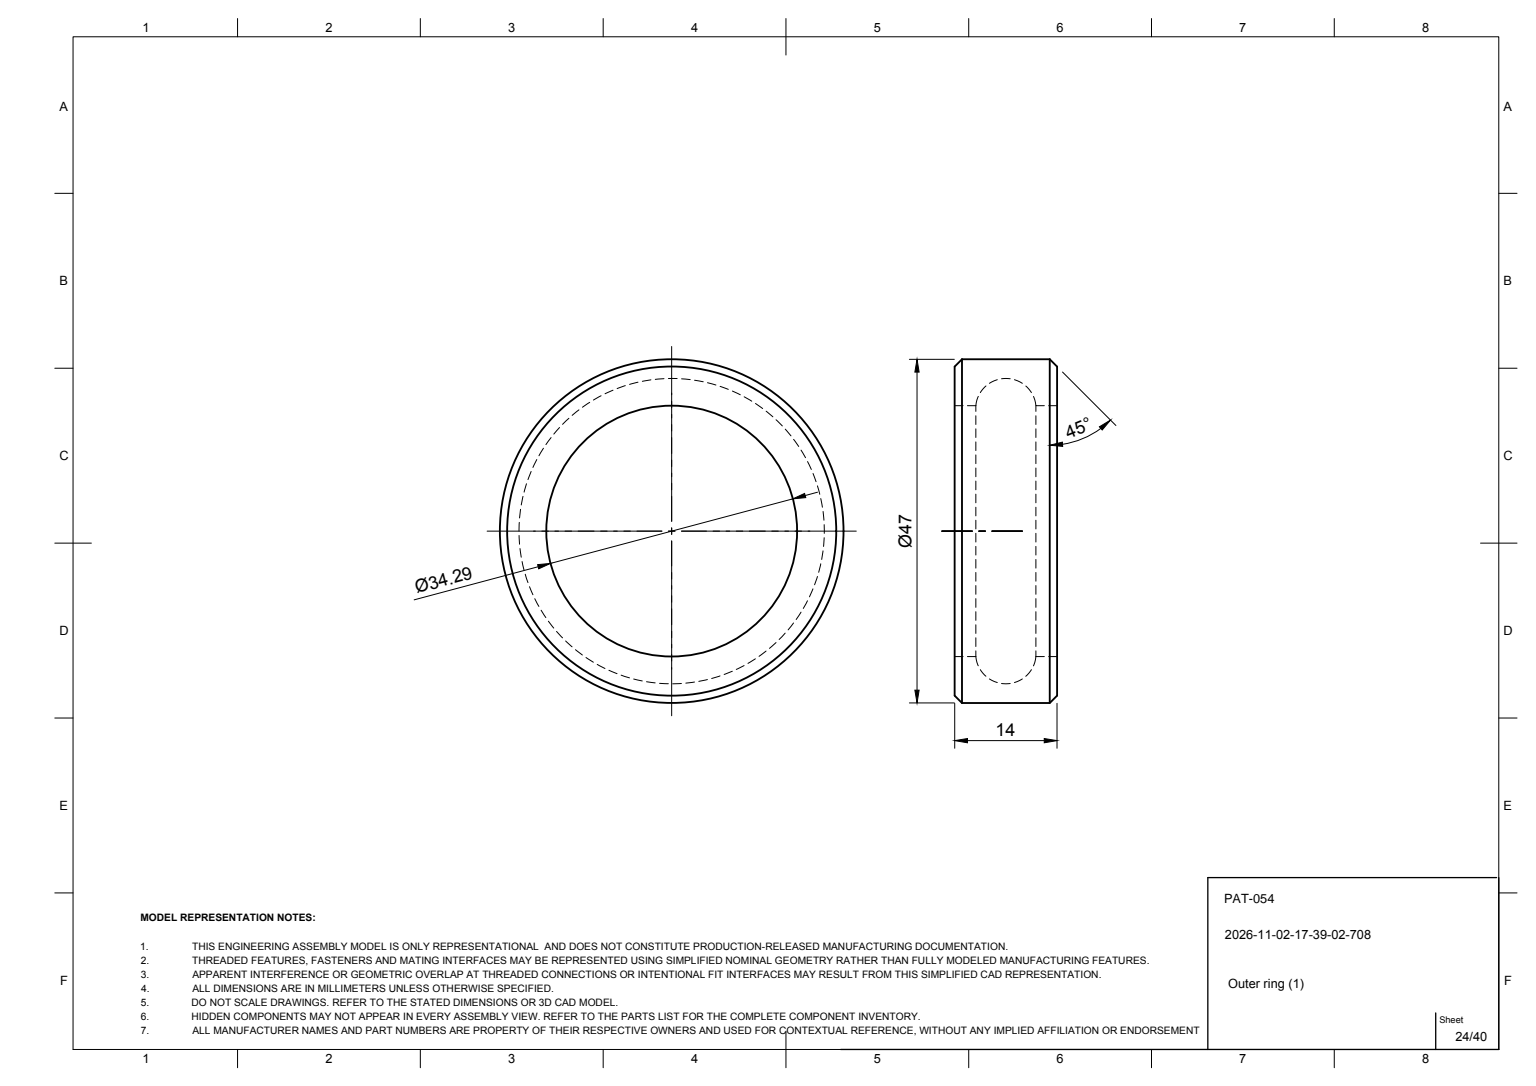
ISO-10303-21;
HEADER;
/* Generated by software containing ST-Developer
 * from STEP Tools, Inc. (www.steptools.com) 
 */

FILE_DESCRIPTION(
/* description */ ('PAT-054'),
/* implementation_level */ '2;1');

FILE_NAME(
/* name */ 'Outer ring (1).step',
/* time_stamp */ '2026-10-29T16:38:13-07:00',
/* author */ (''),
/* organization */ (''),
/* preprocessor_version */ 'ST-DEVELOPER v20.2',
/* originating_system */ 'Autodesk Translation Framework v15.17.0.0',
/* authorisation */ '');

FILE_SCHEMA (('AUTOMOTIVE_DESIGN { 1 0 10303 214 3 1 1 }'));
ENDSEC;

DATA;
#10=MECHANICAL_DESIGN_GEOMETRIC_PRESENTATION_REPRESENTATION('',(#921),#33981);
#783=CONICAL_SURFACE('',#14032,2.3,0.785398163397449);
#784=CONICAL_SURFACE('',#14036,2.3,0.785398163397449);
#810=TOROIDAL_SURFACE('',#14021,1.675,0.412776);
#826=SHAPE_REPRESENTATION_RELATIONSHIP('SRR','None',#34201,#870);
#870=ADVANCED_BREP_SHAPE_REPRESENTATION('',(#980),#33949);
#921=STYLED_ITEM('',(#34517),#980);
#980=MANIFOLD_SOLID_BREP('Body1',#13032);
#1139=FACE_BOUND('',#2637,.T.);
#1140=FACE_BOUND('',#2642,.T.);
#1329=PLANE('',#14029);
#1330=PLANE('',#14038);
#1784=FACE_OUTER_BOUND('',#2634,.T.);
#1785=FACE_OUTER_BOUND('',#2635,.T.);
#1786=FACE_OUTER_BOUND('',#2636,.T.);
#1787=FACE_OUTER_BOUND('',#2638,.T.);
#1788=FACE_OUTER_BOUND('',#2639,.T.);
#1789=FACE_OUTER_BOUND('',#2640,.T.);
#1790=FACE_OUTER_BOUND('',#2641,.T.);
#1791=FACE_OUTER_BOUND('',#2643,.T.);
#2634=EDGE_LOOP('',(#9457,#9458,#9459,#9460,#9461,#9462));
#2635=EDGE_LOOP('',(#9463,#9464,#9465,#9466,#9467));
#2636=EDGE_LOOP('',(#9468));
#2637=EDGE_LOOP('',(#9469));
#2638=EDGE_LOOP('',(#9470,#9471,#9472,#9473));
#2639=EDGE_LOOP('',(#9474,#9475,#9476,#9477));
#2640=EDGE_LOOP('',(#9478,#9479,#9480,#9481));
#2641=EDGE_LOOP('',(#9482));
#2642=EDGE_LOOP('',(#9483));
#2643=EDGE_LOOP('',(#9484,#9485,#9486,#9487,#9488));
#3479=LINE('',#19841,#4413);
#3480=LINE('',#19850,#4414);
#3481=LINE('',#19854,#4415);
#3482=LINE('',#19858,#4416);
#3483=LINE('',#19861,#4417);
#4413=VECTOR('',#16072,1.71469);
#4414=VECTOR('',#16083,2.3);
#4415=VECTOR('',#16088,2.35);
#4416=VECTOR('',#16093,2.3);
#4417=VECTOR('',#16098,1.71469);
#5333=CIRCLE('',#14022,1.71469);
#5334=CIRCLE('',#14023,1.71469);
#5335=CIRCLE('',#14024,0.412776);
#5336=CIRCLE('',#14025,1.71469);
#5337=CIRCLE('',#14026,1.71469);
#5338=CIRCLE('',#14028,1.71469);
#5339=CIRCLE('',#14030,2.25);
#5340=CIRCLE('',#14031,1.71469);
#5341=CIRCLE('',#14033,2.35);
#5342=CIRCLE('',#14035,2.35);
#5343=CIRCLE('',#14037,2.25);
#5900=VERTEX_POINT('',#19829);
#5901=VERTEX_POINT('',#19830);
#5902=VERTEX_POINT('',#19833);
#5903=VERTEX_POINT('',#19835);
#5904=VERTEX_POINT('',#19839);
#5905=VERTEX_POINT('',#19843);
#5906=VERTEX_POINT('',#19845);
#5907=VERTEX_POINT('',#19848);
#5908=VERTEX_POINT('',#19852);
#5909=VERTEX_POINT('',#19856);
#7228=EDGE_CURVE('',#5900,#5901,#5333,.T.);
#7229=EDGE_CURVE('',#5901,#5900,#5334,.T.);
#7230=EDGE_CURVE('',#5901,#5902,#5335,.T.);
#7231=EDGE_CURVE('',#5903,#5902,#5336,.T.);
#7232=EDGE_CURVE('',#5902,#5903,#5337,.T.);
#7233=EDGE_CURVE('',#5904,#5904,#5338,.T.);
#7234=EDGE_CURVE('',#5904,#5903,#3479,.T.);
#7235=EDGE_CURVE('',#5905,#5905,#5339,.T.);
#7236=EDGE_CURVE('',#5906,#5906,#5340,.T.);
#7237=EDGE_CURVE('',#5907,#5907,#5341,.T.);
#7238=EDGE_CURVE('',#5907,#5905,#3480,.T.);
#7239=EDGE_CURVE('',#5908,#5908,#5342,.T.);
#7240=EDGE_CURVE('',#5908,#5907,#3481,.T.);
#7241=EDGE_CURVE('',#5909,#5909,#5343,.T.);
#7242=EDGE_CURVE('',#5909,#5908,#3482,.T.);
#7243=EDGE_CURVE('',#5900,#5906,#3483,.T.);
#9457=ORIENTED_EDGE('',*,*,#7228,.F.);
#9458=ORIENTED_EDGE('',*,*,#7229,.F.);
#9459=ORIENTED_EDGE('',*,*,#7230,.T.);
#9460=ORIENTED_EDGE('',*,*,#7231,.F.);
#9461=ORIENTED_EDGE('',*,*,#7232,.F.);
#9462=ORIENTED_EDGE('',*,*,#7230,.F.);
#9463=ORIENTED_EDGE('',*,*,#7233,.T.);
#9464=ORIENTED_EDGE('',*,*,#7234,.T.);
#9465=ORIENTED_EDGE('',*,*,#7231,.T.);
#9466=ORIENTED_EDGE('',*,*,#7232,.T.);
#9467=ORIENTED_EDGE('',*,*,#7234,.F.);
#9468=ORIENTED_EDGE('',*,*,#7235,.F.);
#9469=ORIENTED_EDGE('',*,*,#7236,.T.);
#9470=ORIENTED_EDGE('',*,*,#7237,.F.);
#9471=ORIENTED_EDGE('',*,*,#7238,.T.);
#9472=ORIENTED_EDGE('',*,*,#7235,.T.);
#9473=ORIENTED_EDGE('',*,*,#7238,.F.);
#9474=ORIENTED_EDGE('',*,*,#7239,.F.);
#9475=ORIENTED_EDGE('',*,*,#7240,.T.);
#9476=ORIENTED_EDGE('',*,*,#7237,.T.);
#9477=ORIENTED_EDGE('',*,*,#7240,.F.);
#9478=ORIENTED_EDGE('',*,*,#7241,.F.);
#9479=ORIENTED_EDGE('',*,*,#7242,.T.);
#9480=ORIENTED_EDGE('',*,*,#7239,.T.);
#9481=ORIENTED_EDGE('',*,*,#7242,.F.);
#9482=ORIENTED_EDGE('',*,*,#7241,.T.);
#9483=ORIENTED_EDGE('',*,*,#7233,.F.);
#9484=ORIENTED_EDGE('',*,*,#7228,.T.);
#9485=ORIENTED_EDGE('',*,*,#7229,.T.);
#9486=ORIENTED_EDGE('',*,*,#7243,.T.);
#9487=ORIENTED_EDGE('',*,*,#7236,.F.);
#9488=ORIENTED_EDGE('',*,*,#7243,.F.);
#12064=CYLINDRICAL_SURFACE('',#14027,1.71469);
#12065=CYLINDRICAL_SURFACE('',#14034,2.35);
#12066=CYLINDRICAL_SURFACE('',#14039,1.71469);
#12496=ADVANCED_FACE('',(#1784),#810,.F.);
#12497=ADVANCED_FACE('',(#1785),#12064,.F.);
#12498=ADVANCED_FACE('',(#1786,#1139),#1329,.T.);
#12499=ADVANCED_FACE('',(#1787),#783,.T.);
#12500=ADVANCED_FACE('',(#1788),#12065,.T.);
#12501=ADVANCED_FACE('',(#1789),#784,.T.);
#12502=ADVANCED_FACE('',(#1790,#1140),#1330,.T.);
#12503=ADVANCED_FACE('',(#1791),#12066,.F.);
#13032=CLOSED_SHELL('',(#12496,#12497,#12498,#12499,#12500,#12501,#12502,
#12503));
#14020=AXIS2_PLACEMENT_3D('',#19827,#16054,#16055);
#14021=AXIS2_PLACEMENT_3D('',#19828,#16056,#16057);
#14022=AXIS2_PLACEMENT_3D('',#19831,#16058,#16059);
#14023=AXIS2_PLACEMENT_3D('',#19832,#16060,#16061);
#14024=AXIS2_PLACEMENT_3D('',#19834,#16062,#16063);
#14025=AXIS2_PLACEMENT_3D('',#19836,#16064,#16065);
#14026=AXIS2_PLACEMENT_3D('',#19837,#16066,#16067);
#14027=AXIS2_PLACEMENT_3D('',#19838,#16068,#16069);
#14028=AXIS2_PLACEMENT_3D('',#19840,#16070,#16071);
#14029=AXIS2_PLACEMENT_3D('',#19842,#16073,#16074);
#14030=AXIS2_PLACEMENT_3D('',#19844,#16075,#16076);
#14031=AXIS2_PLACEMENT_3D('',#19846,#16077,#16078);
#14032=AXIS2_PLACEMENT_3D('',#19847,#16079,#16080);
#14033=AXIS2_PLACEMENT_3D('',#19849,#16081,#16082);
#14034=AXIS2_PLACEMENT_3D('',#19851,#16084,#16085);
#14035=AXIS2_PLACEMENT_3D('',#19853,#16086,#16087);
#14036=AXIS2_PLACEMENT_3D('',#19855,#16089,#16090);
#14037=AXIS2_PLACEMENT_3D('',#19857,#16091,#16092);
#14038=AXIS2_PLACEMENT_3D('',#19859,#16094,#16095);
#14039=AXIS2_PLACEMENT_3D('',#19860,#16096,#16097);
#16054=DIRECTION('axis',(0.,0.,1.));
#16055=DIRECTION('refdir',(1.,0.,0.));
#16056=DIRECTION('center_axis',(0.,-1.,0.));
#16057=DIRECTION('ref_axis',(0.,0.,-1.));
#16058=DIRECTION('center_axis',(0.,-1.,0.));
#16059=DIRECTION('ref_axis',(1.,0.,0.));
#16060=DIRECTION('center_axis',(0.,-1.,0.));
#16061=DIRECTION('ref_axis',(1.,0.,0.));
#16062=DIRECTION('center_axis',(1.,0.,1.22464679914735E-16));
#16063=DIRECTION('ref_axis',(-1.22464679914735E-16,0.,1.));
#16064=DIRECTION('center_axis',(0.,1.,0.));
#16065=DIRECTION('ref_axis',(1.,0.,0.));
#16066=DIRECTION('center_axis',(0.,1.,0.));
#16067=DIRECTION('ref_axis',(1.,0.,0.));
#16068=DIRECTION('center_axis',(0.,-1.,0.));
#16069=DIRECTION('ref_axis',(1.,0.,0.));
#16070=DIRECTION('center_axis',(0.,-1.,0.));
#16071=DIRECTION('ref_axis',(1.,0.,0.));
#16072=DIRECTION('',(0.,1.,0.));
#16073=DIRECTION('center_axis',(0.,1.,0.));
#16074=DIRECTION('ref_axis',(0.,0.,1.));
#16075=DIRECTION('center_axis',(0.,-1.,0.));
#16076=DIRECTION('ref_axis',(1.,0.,0.));
#16077=DIRECTION('center_axis',(0.,-1.,0.));
#16078=DIRECTION('ref_axis',(1.,0.,0.));
#16079=DIRECTION('center_axis',(0.,-1.,0.));
#16080=DIRECTION('ref_axis',(1.,0.,0.));
#16081=DIRECTION('center_axis',(0.,-1.,0.));
#16082=DIRECTION('ref_axis',(1.,0.,0.));
#16083=DIRECTION('',(0.707106781186548,0.707106781186547,8.65956056235494E-17));
#16084=DIRECTION('center_axis',(0.,-1.,0.));
#16085=DIRECTION('ref_axis',(1.,0.,0.));
#16086=DIRECTION('center_axis',(0.,-1.,0.));
#16087=DIRECTION('ref_axis',(1.,0.,0.));
#16088=DIRECTION('',(0.,1.,0.));
#16089=DIRECTION('center_axis',(0.,1.,0.));
#16090=DIRECTION('ref_axis',(1.,0.,0.));
#16091=DIRECTION('center_axis',(0.,-1.,0.));
#16092=DIRECTION('ref_axis',(1.,0.,0.));
#16093=DIRECTION('',(-0.707106781186548,0.707106781186547,-8.65956056235494E-17));
#16094=DIRECTION('center_axis',(0.,-1.,0.));
#16095=DIRECTION('ref_axis',(0.,0.,-1.));
#16096=DIRECTION('center_axis',(0.,-1.,0.));
#16097=DIRECTION('ref_axis',(1.,0.,0.));
#16098=DIRECTION('',(0.,1.,0.));
#19827=CARTESIAN_POINT('',(0.,0.,0.));
#19828=CARTESIAN_POINT('Origin',(0.,0.,0.));
#19829=CARTESIAN_POINT('',(-1.71469,0.410863395882378,-2.09988962002998E-16));
#19830=CARTESIAN_POINT('',(-2.09988962002998E-16,0.410863395882378,1.71469));
#19831=CARTESIAN_POINT('Origin',(0.,0.410863395882378,0.));
#19832=CARTESIAN_POINT('Origin',(0.,0.410863395882378,0.));
#19833=CARTESIAN_POINT('',(-2.09988962002998E-16,-0.410863395882378,1.71469));
#19834=CARTESIAN_POINT('Origin',(-2.05128338857182E-16,0.,1.675));
#19835=CARTESIAN_POINT('',(-1.71469,-0.410863395882378,2.09988962002998E-16));
#19836=CARTESIAN_POINT('Origin',(0.,-0.410863395882378,0.));
#19837=CARTESIAN_POINT('Origin',(0.,-0.410863395882378,0.));
#19838=CARTESIAN_POINT('Origin',(0.,0.,0.));
#19839=CARTESIAN_POINT('',(-1.71469,-0.7,-2.09988962002998E-16));
#19840=CARTESIAN_POINT('Origin',(0.,-0.7,0.));
#19841=CARTESIAN_POINT('',(-1.71469,0.,-2.09988962002998E-16));
#19842=CARTESIAN_POINT('Origin',(2.25,0.7,0.));
#19843=CARTESIAN_POINT('',(-2.25,0.7,-2.75545529808154E-16));
#19844=CARTESIAN_POINT('Origin',(0.,0.7,0.));
#19845=CARTESIAN_POINT('',(-1.71469,0.7,-2.09988962002998E-16));
#19846=CARTESIAN_POINT('Origin',(0.,0.7,0.));
#19847=CARTESIAN_POINT('Origin',(0.,0.65,0.));
#19848=CARTESIAN_POINT('',(-2.35,0.6,-2.87791997799628E-16));
#19849=CARTESIAN_POINT('Origin',(0.,0.6,0.));
#19850=CARTESIAN_POINT('',(-2.3,0.65,-2.81668763803891E-16));
#19851=CARTESIAN_POINT('Origin',(0.,0.,0.));
#19852=CARTESIAN_POINT('',(-2.35,-0.6,-2.87791997799628E-16));
#19853=CARTESIAN_POINT('Origin',(0.,-0.6,0.));
#19854=CARTESIAN_POINT('',(-2.35,0.,-2.87791997799628E-16));
#19855=CARTESIAN_POINT('Origin',(0.,-0.65,0.));
#19856=CARTESIAN_POINT('',(-2.25,-0.7,-2.75545529808154E-16));
#19857=CARTESIAN_POINT('Origin',(0.,-0.7,0.));
#19858=CARTESIAN_POINT('',(-2.3,-0.65,-2.81668763803891E-16));
#19859=CARTESIAN_POINT('Origin',(1.71469,-0.7,0.));
#19860=CARTESIAN_POINT('Origin',(0.,0.,0.));
#19861=CARTESIAN_POINT('',(-1.71469,0.,-2.09988962002998E-16));
#33897=UNCERTAINTY_MEASURE_WITH_UNIT(LENGTH_MEASURE(0.001),#33982,
'DISTANCE_ACCURACY_VALUE',
'Maximum model space distance between geometric entities at asserted c
onnectivities');
#33929=UNCERTAINTY_MEASURE_WITH_UNIT(LENGTH_MEASURE(0.001),#33982,
'DISTANCE_ACCURACY_VALUE',
'Maximum model space distance between geometric entities at asserted c
onnectivities');
#33949=(
GEOMETRIC_REPRESENTATION_CONTEXT(3)
GLOBAL_UNCERTAINTY_ASSIGNED_CONTEXT((#33897))
GLOBAL_UNIT_ASSIGNED_CONTEXT((#33982,#33984,#33985))
REPRESENTATION_CONTEXT('','3D')
);
#33981=(
GEOMETRIC_REPRESENTATION_CONTEXT(3)
GLOBAL_UNCERTAINTY_ASSIGNED_CONTEXT((#33929))
GLOBAL_UNIT_ASSIGNED_CONTEXT((#33982,#33984,#33985))
REPRESENTATION_CONTEXT('','3D')
);
#33982=(
LENGTH_UNIT()
NAMED_UNIT(*)
SI_UNIT(.CENTI.,.METRE.)
);
#33984=(
NAMED_UNIT(*)
PLANE_ANGLE_UNIT()
SI_UNIT($,.RADIAN.)
);
#33985=(
NAMED_UNIT(*)
SI_UNIT($,.STERADIAN.)
SOLID_ANGLE_UNIT()
);
#34005=SHAPE_DEFINITION_REPRESENTATION(#34061,#34201);
#34061=PRODUCT_DEFINITION_SHAPE('',$,#34253);
#34201=SHAPE_REPRESENTATION('',(#14020),#33949);
#34233=PRODUCT_DEFINITION_CONTEXT('part definition',#34388,'design');
#34253=PRODUCT_DEFINITION('Outer ring (1)','Outer ring (1)',#34304,#34233);
#34304=PRODUCT_DEFINITION_FORMATION('',$,#34409);
#34388=APPLICATION_CONTEXT(
'Core Data for Automotive Mechanical Design Process');
#34389=PRODUCT_CONTEXT('part definition',#34388,'mechanical');
#34409=PRODUCT('Outer ring (1)','Outer ring (1)','Outer ring (1)',(#34389));
#34511=COLOUR_RGB('Grey',0.48,0.52,0.57);
#34512=FILL_AREA_STYLE_COLOUR('',#34511);
#34513=FILL_AREA_STYLE('',(#34512));
#34514=SURFACE_STYLE_FILL_AREA(#34513);
#34515=SURFACE_SIDE_STYLE('',(#34514));
#34516=SURFACE_STYLE_USAGE(.BOTH.,#34515);
#34517=PRESENTATION_STYLE_ASSIGNMENT((#34516));
ENDSEC;
END-ISO-10303-21;
